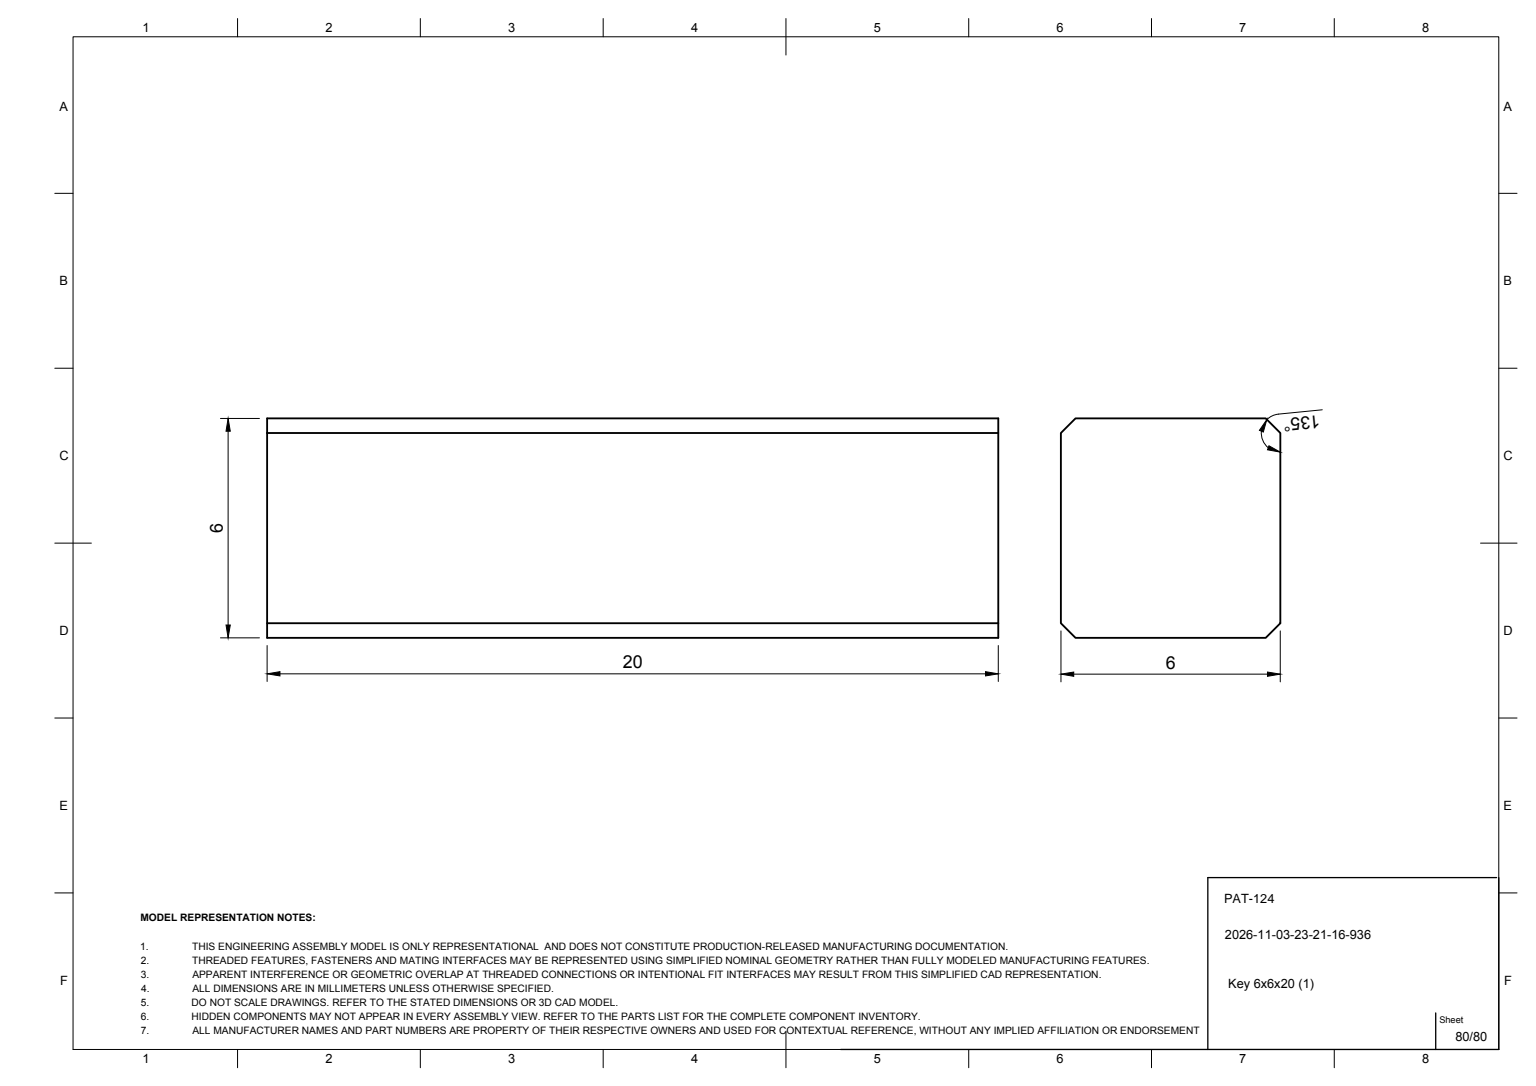
ISO-10303-21;
HEADER;
/* Generated by software containing ST-Developer
 * from STEP Tools, Inc. (www.steptools.com) 
 */

FILE_DESCRIPTION(
/* description */ ('XY cross-slide table'),
/* implementation_level */ '2;1');

FILE_NAME(
/* name */ 'Key 6x6x20 (1).step',
/* time_stamp */ '2026-10-28T03:22:46-07:00',
/* author */ (''),
/* organization */ (''),
/* preprocessor_version */ 'ST-DEVELOPER v20.2',
/* originating_system */ 'Autodesk Translation Framework v15.17.0.0',
/* authorisation */ '');

FILE_SCHEMA (('AUTOMOTIVE_DESIGN { 1 0 10303 214 3 1 1 }'));
ENDSEC;

DATA;
#10=MECHANICAL_DESIGN_GEOMETRIC_PRESENTATION_REPRESENTATION('',(#1779),#62984);
#1583=SHAPE_REPRESENTATION_RELATIONSHIP('SRR','None',#63443,#1666);
#1666=ADVANCED_BREP_SHAPE_REPRESENTATION('',(#1884),#62980);
#1779=STYLED_ITEM('',(#63912),#1884);
#1884=MANIFOLD_SOLID_BREP('Body1',#23081);
#2837=PLANE('',#26348);
#2838=PLANE('',#26349);
#2839=PLANE('',#26350);
#2840=PLANE('',#26351);
#2841=PLANE('',#26352);
#2842=PLANE('',#26353);
#2843=PLANE('',#26354);
#2844=PLANE('',#26355);
#2845=PLANE('',#26356);
#2846=PLANE('',#26357);
#4140=FACE_OUTER_BOUND('',#5859,.T.);
#4141=FACE_OUTER_BOUND('',#5860,.T.);
#4142=FACE_OUTER_BOUND('',#5861,.T.);
#4143=FACE_OUTER_BOUND('',#5862,.T.);
#4144=FACE_OUTER_BOUND('',#5863,.T.);
#4145=FACE_OUTER_BOUND('',#5864,.T.);
#4146=FACE_OUTER_BOUND('',#5865,.T.);
#4147=FACE_OUTER_BOUND('',#5866,.T.);
#4148=FACE_OUTER_BOUND('',#5867,.T.);
#4149=FACE_OUTER_BOUND('',#5868,.T.);
#5859=EDGE_LOOP('',(#20866,#20867,#20868,#20869,#20870,#20871,#20872,#20873));
#5860=EDGE_LOOP('',(#20874,#20875,#20876,#20877));
#5861=EDGE_LOOP('',(#20878,#20879,#20880,#20881));
#5862=EDGE_LOOP('',(#20882,#20883,#20884,#20885));
#5863=EDGE_LOOP('',(#20886,#20887,#20888,#20889));
#5864=EDGE_LOOP('',(#20890,#20891,#20892,#20893,#20894,#20895,#20896,#20897));
#5865=EDGE_LOOP('',(#20898,#20899,#20900,#20901));
#5866=EDGE_LOOP('',(#20902,#20903,#20904,#20905));
#5867=EDGE_LOOP('',(#20906,#20907,#20908,#20909));
#5868=EDGE_LOOP('',(#20910,#20911,#20912,#20913));
#7322=LINE('',#62550,#8809);
#7323=LINE('',#62552,#8810);
#7324=LINE('',#62554,#8811);
#7325=LINE('',#62556,#8812);
#7326=LINE('',#62558,#8813);
#7327=LINE('',#62560,#8814);
#7328=LINE('',#62562,#8815);
#7329=LINE('',#62563,#8816);
#7330=LINE('',#62566,#8817);
#7331=LINE('',#62568,#8818);
#7332=LINE('',#62569,#8819);
#7333=LINE('',#62572,#8820);
#7334=LINE('',#62573,#8821);
#7335=LINE('',#62576,#8822);
#7336=LINE('',#62577,#8823);
#7337=LINE('',#62580,#8824);
#7338=LINE('',#62581,#8825);
#7339=LINE('',#62585,#8826);
#7340=LINE('',#62586,#8827);
#7341=LINE('',#62588,#8828);
#7342=LINE('',#62589,#8829);
#7343=LINE('',#62591,#8830);
#7344=LINE('',#62593,#8831);
#7345=LINE('',#62595,#8832);
#8809=VECTOR('',#32575,1.);
#8810=VECTOR('',#32576,1.);
#8811=VECTOR('',#32577,1.);
#8812=VECTOR('',#32578,1.);
#8813=VECTOR('',#32579,1.);
#8814=VECTOR('',#32580,1.);
#8815=VECTOR('',#32581,1.);
#8816=VECTOR('',#32582,1.);
#8817=VECTOR('',#32585,1.);
#8818=VECTOR('',#32586,1.);
#8819=VECTOR('',#32587,1.);
#8820=VECTOR('',#32590,1.);
#8821=VECTOR('',#32591,1.);
#8822=VECTOR('',#32594,1.);
#8823=VECTOR('',#32595,1.);
#8824=VECTOR('',#32598,1.);
#8825=VECTOR('',#32599,1.);
#8826=VECTOR('',#32602,1.);
#8827=VECTOR('',#32603,1.);
#8828=VECTOR('',#32604,1.);
#8829=VECTOR('',#32605,1.);
#8830=VECTOR('',#32608,1.);
#8831=VECTOR('',#32611,1.);
#8832=VECTOR('',#32614,1.);
#11780=VERTEX_POINT('',#62548);
#11781=VERTEX_POINT('',#62549);
#11782=VERTEX_POINT('',#62551);
#11783=VERTEX_POINT('',#62553);
#11784=VERTEX_POINT('',#62555);
#11785=VERTEX_POINT('',#62557);
#11786=VERTEX_POINT('',#62559);
#11787=VERTEX_POINT('',#62561);
#11788=VERTEX_POINT('',#62565);
#11789=VERTEX_POINT('',#62567);
#11790=VERTEX_POINT('',#62571);
#11791=VERTEX_POINT('',#62575);
#11792=VERTEX_POINT('',#62579);
#11793=VERTEX_POINT('',#62583);
#11794=VERTEX_POINT('',#62584);
#11795=VERTEX_POINT('',#62587);
#14817=EDGE_CURVE('',#11780,#11781,#7322,.T.);
#14818=EDGE_CURVE('',#11782,#11780,#7323,.T.);
#14819=EDGE_CURVE('',#11783,#11782,#7324,.T.);
#14820=EDGE_CURVE('',#11784,#11783,#7325,.T.);
#14821=EDGE_CURVE('',#11785,#11784,#7326,.T.);
#14822=EDGE_CURVE('',#11786,#11785,#7327,.T.);
#14823=EDGE_CURVE('',#11787,#11786,#7328,.T.);
#14824=EDGE_CURVE('',#11781,#11787,#7329,.T.);
#14825=EDGE_CURVE('',#11784,#11788,#7330,.T.);
#14826=EDGE_CURVE('',#11788,#11789,#7331,.T.);
#14827=EDGE_CURVE('',#11789,#11785,#7332,.T.);
#14828=EDGE_CURVE('',#11790,#11783,#7333,.T.);
#14829=EDGE_CURVE('',#11790,#11788,#7334,.T.);
#14830=EDGE_CURVE('',#11782,#11791,#7335,.T.);
#14831=EDGE_CURVE('',#11791,#11790,#7336,.T.);
#14832=EDGE_CURVE('',#11792,#11780,#7337,.T.);
#14833=EDGE_CURVE('',#11792,#11791,#7338,.T.);
#14834=EDGE_CURVE('',#11793,#11794,#7339,.T.);
#14835=EDGE_CURVE('',#11789,#11793,#7340,.T.);
#14836=EDGE_CURVE('',#11795,#11792,#7341,.T.);
#14837=EDGE_CURVE('',#11794,#11795,#7342,.T.);
#14838=EDGE_CURVE('',#11786,#11793,#7343,.T.);
#14839=EDGE_CURVE('',#11781,#11795,#7344,.T.);
#14840=EDGE_CURVE('',#11794,#11787,#7345,.T.);
#20866=ORIENTED_EDGE('',*,*,#14817,.F.);
#20867=ORIENTED_EDGE('',*,*,#14818,.F.);
#20868=ORIENTED_EDGE('',*,*,#14819,.F.);
#20869=ORIENTED_EDGE('',*,*,#14820,.F.);
#20870=ORIENTED_EDGE('',*,*,#14821,.F.);
#20871=ORIENTED_EDGE('',*,*,#14822,.F.);
#20872=ORIENTED_EDGE('',*,*,#14823,.F.);
#20873=ORIENTED_EDGE('',*,*,#14824,.F.);
#20874=ORIENTED_EDGE('',*,*,#14821,.T.);
#20875=ORIENTED_EDGE('',*,*,#14825,.T.);
#20876=ORIENTED_EDGE('',*,*,#14826,.T.);
#20877=ORIENTED_EDGE('',*,*,#14827,.T.);
#20878=ORIENTED_EDGE('',*,*,#14820,.T.);
#20879=ORIENTED_EDGE('',*,*,#14828,.F.);
#20880=ORIENTED_EDGE('',*,*,#14829,.T.);
#20881=ORIENTED_EDGE('',*,*,#14825,.F.);
#20882=ORIENTED_EDGE('',*,*,#14819,.T.);
#20883=ORIENTED_EDGE('',*,*,#14830,.T.);
#20884=ORIENTED_EDGE('',*,*,#14831,.T.);
#20885=ORIENTED_EDGE('',*,*,#14828,.T.);
#20886=ORIENTED_EDGE('',*,*,#14818,.T.);
#20887=ORIENTED_EDGE('',*,*,#14832,.F.);
#20888=ORIENTED_EDGE('',*,*,#14833,.T.);
#20889=ORIENTED_EDGE('',*,*,#14830,.F.);
#20890=ORIENTED_EDGE('',*,*,#14834,.F.);
#20891=ORIENTED_EDGE('',*,*,#14835,.F.);
#20892=ORIENTED_EDGE('',*,*,#14826,.F.);
#20893=ORIENTED_EDGE('',*,*,#14829,.F.);
#20894=ORIENTED_EDGE('',*,*,#14831,.F.);
#20895=ORIENTED_EDGE('',*,*,#14833,.F.);
#20896=ORIENTED_EDGE('',*,*,#14836,.F.);
#20897=ORIENTED_EDGE('',*,*,#14837,.F.);
#20898=ORIENTED_EDGE('',*,*,#14822,.T.);
#20899=ORIENTED_EDGE('',*,*,#14827,.F.);
#20900=ORIENTED_EDGE('',*,*,#14835,.T.);
#20901=ORIENTED_EDGE('',*,*,#14838,.F.);
#20902=ORIENTED_EDGE('',*,*,#14817,.T.);
#20903=ORIENTED_EDGE('',*,*,#14839,.T.);
#20904=ORIENTED_EDGE('',*,*,#14836,.T.);
#20905=ORIENTED_EDGE('',*,*,#14832,.T.);
#20906=ORIENTED_EDGE('',*,*,#14823,.T.);
#20907=ORIENTED_EDGE('',*,*,#14838,.T.);
#20908=ORIENTED_EDGE('',*,*,#14834,.T.);
#20909=ORIENTED_EDGE('',*,*,#14840,.T.);
#20910=ORIENTED_EDGE('',*,*,#14824,.T.);
#20911=ORIENTED_EDGE('',*,*,#14840,.F.);
#20912=ORIENTED_EDGE('',*,*,#14837,.T.);
#20913=ORIENTED_EDGE('',*,*,#14839,.F.);
#22921=ADVANCED_FACE('',(#4140),#2837,.F.);
#22922=ADVANCED_FACE('',(#4141),#2838,.T.);
#22923=ADVANCED_FACE('',(#4142),#2839,.T.);
#22924=ADVANCED_FACE('',(#4143),#2840,.T.);
#22925=ADVANCED_FACE('',(#4144),#2841,.T.);
#22926=ADVANCED_FACE('',(#4145),#2842,.T.);
#22927=ADVANCED_FACE('',(#4146),#2843,.F.);
#22928=ADVANCED_FACE('',(#4147),#2844,.T.);
#22929=ADVANCED_FACE('',(#4148),#2845,.T.);
#22930=ADVANCED_FACE('',(#4149),#2846,.T.);
#23081=CLOSED_SHELL('',(#22921,#22922,#22923,#22924,#22925,#22926,#22927,
#22928,#22929,#22930));
#26347=AXIS2_PLACEMENT_3D('',#62546,#32571,#32572);
#26348=AXIS2_PLACEMENT_3D('',#62547,#32573,#32574);
#26349=AXIS2_PLACEMENT_3D('',#62564,#32583,#32584);
#26350=AXIS2_PLACEMENT_3D('',#62570,#32588,#32589);
#26351=AXIS2_PLACEMENT_3D('',#62574,#32592,#32593);
#26352=AXIS2_PLACEMENT_3D('',#62578,#32596,#32597);
#26353=AXIS2_PLACEMENT_3D('',#62582,#32600,#32601);
#26354=AXIS2_PLACEMENT_3D('',#62590,#32606,#32607);
#26355=AXIS2_PLACEMENT_3D('',#62592,#32609,#32610);
#26356=AXIS2_PLACEMENT_3D('',#62594,#32612,#32613);
#26357=AXIS2_PLACEMENT_3D('',#62596,#32615,#32616);
#32571=DIRECTION('axis',(0.,0.,1.));
#32572=DIRECTION('refdir',(1.,0.,0.));
#32573=DIRECTION('center_axis',(1.,0.,0.));
#32574=DIRECTION('ref_axis',(0.,0.,-1.));
#32575=DIRECTION('',(0.,-0.707106781186547,-0.707106781186548));
#32576=DIRECTION('',(0.,-1.,0.));
#32577=DIRECTION('',(0.,-0.707106781186547,0.707106781186548));
#32578=DIRECTION('',(0.,0.,1.));
#32579=DIRECTION('',(0.,0.707106781186547,0.707106781186548));
#32580=DIRECTION('',(0.,1.,0.));
#32581=DIRECTION('',(0.,0.707106781186547,-0.707106781186548));
#32582=DIRECTION('',(0.,0.,-1.));
#32583=DIRECTION('center_axis',(0.,0.707106781186548,-0.707106781186547));
#32584=DIRECTION('ref_axis',(-1.,0.,0.));
#32585=DIRECTION('',(1.,0.,0.));
#32586=DIRECTION('',(0.,-0.707106781186547,-0.707106781186548));
#32587=DIRECTION('',(-1.,0.,0.));
#32588=DIRECTION('center_axis',(0.,1.,0.));
#32589=DIRECTION('ref_axis',(-1.,0.,0.));
#32590=DIRECTION('',(-1.,0.,0.));
#32591=DIRECTION('',(0.,0.,-1.));
#32592=DIRECTION('center_axis',(0.,0.707106781186548,0.707106781186547));
#32593=DIRECTION('ref_axis',(1.,0.,0.));
#32594=DIRECTION('',(1.,0.,0.));
#32595=DIRECTION('',(0.,0.707106781186547,-0.707106781186548));
#32596=DIRECTION('center_axis',(0.,0.,1.));
#32597=DIRECTION('ref_axis',(1.,0.,0.));
#32598=DIRECTION('',(-1.,0.,0.));
#32599=DIRECTION('',(0.,1.,0.));
#32600=DIRECTION('center_axis',(1.,0.,0.));
#32601=DIRECTION('ref_axis',(0.,0.,-1.));
#32602=DIRECTION('',(0.,-0.707106781186547,0.707106781186548));
#32603=DIRECTION('',(0.,-1.,0.));
#32604=DIRECTION('',(0.,0.707106781186547,0.707106781186548));
#32605=DIRECTION('',(0.,0.,1.));
#32606=DIRECTION('center_axis',(0.,0.,1.));
#32607=DIRECTION('ref_axis',(1.,0.,0.));
#32608=DIRECTION('',(1.,0.,0.));
#32609=DIRECTION('center_axis',(0.,-0.707106781186548,0.707106781186547));
#32610=DIRECTION('ref_axis',(1.,0.,0.));
#32611=DIRECTION('',(1.,0.,0.));
#32612=DIRECTION('center_axis',(0.,-0.707106781186548,-0.707106781186547));
#32613=DIRECTION('ref_axis',(-1.,0.,0.));
#32614=DIRECTION('',(-1.,0.,0.));
#32615=DIRECTION('center_axis',(0.,-1.,0.));
#32616=DIRECTION('ref_axis',(1.,0.,0.));
#62546=CARTESIAN_POINT('',(0.,0.,0.));
#62547=CARTESIAN_POINT('Origin',(-1.,0.,0.35));
#62548=CARTESIAN_POINT('',(-1.,-0.26,0.6));
#62549=CARTESIAN_POINT('',(-1.,-0.3,0.56));
#62550=CARTESIAN_POINT('',(-1.,-0.2675,0.5925));
#62551=CARTESIAN_POINT('',(-1.,0.26,0.6));
#62552=CARTESIAN_POINT('',(-1.,0.,0.6));
#62553=CARTESIAN_POINT('',(-1.,0.3,0.56));
#62554=CARTESIAN_POINT('',(-1.,0.2675,0.5925));
#62555=CARTESIAN_POINT('',(-1.,0.3,0.04));
#62556=CARTESIAN_POINT('',(-1.,0.3,0.175));
#62557=CARTESIAN_POINT('',(-1.,0.26,0.));
#62558=CARTESIAN_POINT('',(-1.,0.2925,0.0325));
#62559=CARTESIAN_POINT('',(-1.,-0.26,0.));
#62560=CARTESIAN_POINT('',(-1.,0.,0.));
#62561=CARTESIAN_POINT('',(-1.,-0.3,0.04));
#62562=CARTESIAN_POINT('',(-1.,-0.2925,0.0325));
#62563=CARTESIAN_POINT('',(-1.,-0.3,0.175));
#62564=CARTESIAN_POINT('Origin',(0.75,0.28,0.02));
#62565=CARTESIAN_POINT('',(1.,0.3,0.04));
#62566=CARTESIAN_POINT('',(0.75,0.3,0.04));
#62567=CARTESIAN_POINT('',(1.,0.26,0.));
#62568=CARTESIAN_POINT('',(1.,0.2925,0.0325));
#62569=CARTESIAN_POINT('',(0.75,0.26,0.));
#62570=CARTESIAN_POINT('Origin',(1.5,0.3,0.));
#62571=CARTESIAN_POINT('',(1.,0.3,0.56));
#62572=CARTESIAN_POINT('',(0.75,0.3,0.56));
#62573=CARTESIAN_POINT('',(1.,0.3,0.175));
#62574=CARTESIAN_POINT('Origin',(0.75,0.28,0.58));
#62575=CARTESIAN_POINT('',(1.,0.26,0.6));
#62576=CARTESIAN_POINT('',(0.75,0.26,0.6));
#62577=CARTESIAN_POINT('',(1.,0.2675,0.5925));
#62578=CARTESIAN_POINT('Origin',(0.,0.,0.6));
#62579=CARTESIAN_POINT('',(1.,-0.26,0.6));
#62580=CARTESIAN_POINT('',(-0.75,-0.26,0.6));
#62581=CARTESIAN_POINT('',(1.,0.,0.6));
#62582=CARTESIAN_POINT('Origin',(1.,0.,0.35));
#62583=CARTESIAN_POINT('',(1.,-0.26,0.));
#62584=CARTESIAN_POINT('',(1.,-0.3,0.04));
#62585=CARTESIAN_POINT('',(1.,-0.2925,0.0325));
#62586=CARTESIAN_POINT('',(1.,0.,0.));
#62587=CARTESIAN_POINT('',(1.,-0.3,0.56));
#62588=CARTESIAN_POINT('',(1.,-0.2675,0.5925));
#62589=CARTESIAN_POINT('',(1.,-0.3,0.175));
#62590=CARTESIAN_POINT('Origin',(0.,0.,0.));
#62591=CARTESIAN_POINT('',(-0.75,-0.26,0.));
#62592=CARTESIAN_POINT('Origin',(-0.75,-0.28,0.58));
#62593=CARTESIAN_POINT('',(-0.75,-0.3,0.56));
#62594=CARTESIAN_POINT('Origin',(-0.75,-0.28,0.02));
#62595=CARTESIAN_POINT('',(-0.75,-0.3,0.04));
#62596=CARTESIAN_POINT('Origin',(-1.5,-0.3,0.));
#62881=UNCERTAINTY_MEASURE_WITH_UNIT(LENGTH_MEASURE(0.001),#62985,
'DISTANCE_ACCURACY_VALUE',
'Maximum model space distance between geometric entities at asserted c
onnectivities');
#62885=UNCERTAINTY_MEASURE_WITH_UNIT(LENGTH_MEASURE(0.001),#62985,
'DISTANCE_ACCURACY_VALUE',
'Maximum model space distance between geometric entities at asserted c
onnectivities');
#62980=(
GEOMETRIC_REPRESENTATION_CONTEXT(3)
GLOBAL_UNCERTAINTY_ASSIGNED_CONTEXT((#62881))
GLOBAL_UNIT_ASSIGNED_CONTEXT((#62985,#62987,#62988))
REPRESENTATION_CONTEXT('','3D')
);
#62984=(
GEOMETRIC_REPRESENTATION_CONTEXT(3)
GLOBAL_UNCERTAINTY_ASSIGNED_CONTEXT((#62885))
GLOBAL_UNIT_ASSIGNED_CONTEXT((#62985,#62987,#62988))
REPRESENTATION_CONTEXT('','3D')
);
#62985=(
LENGTH_UNIT()
NAMED_UNIT(*)
SI_UNIT(.CENTI.,.METRE.)
);
#62987=(
NAMED_UNIT(*)
PLANE_ANGLE_UNIT()
SI_UNIT($,.RADIAN.)
);
#62988=(
NAMED_UNIT(*)
SI_UNIT($,.STERADIAN.)
SOLID_ANGLE_UNIT()
);
#63083=SHAPE_DEFINITION_REPRESENTATION(#63294,#63443);
#63294=PRODUCT_DEFINITION_SHAPE('',$,#63542);
#63443=SHAPE_REPRESENTATION('',(#26347),#62980);
#63447=PRODUCT_DEFINITION_CONTEXT('part definition',#63743,'design');
#63542=PRODUCT_DEFINITION('Key 6x6x20 (1)','Key 6x6x20 (1)',#63640,#63447);
#63640=PRODUCT_DEFINITION_FORMATION('',$,#63839);
#63743=APPLICATION_CONTEXT(
'Core Data for Automotive Mechanical Design Process');
#63744=PRODUCT_CONTEXT('part definition',#63743,'mechanical');
#63839=PRODUCT('Key 6x6x20 (1)','Key 6x6x20 (1)','Key 6x6x20 (1)',(#63744));
#63906=COLOUR_RGB('Grey',0.48,0.52,0.57);
#63907=FILL_AREA_STYLE_COLOUR('',#63906);
#63908=FILL_AREA_STYLE('',(#63907));
#63909=SURFACE_STYLE_FILL_AREA(#63908);
#63910=SURFACE_SIDE_STYLE('',(#63909));
#63911=SURFACE_STYLE_USAGE(.BOTH.,#63910);
#63912=PRESENTATION_STYLE_ASSIGNMENT((#63911));
ENDSEC;
END-ISO-10303-21;
